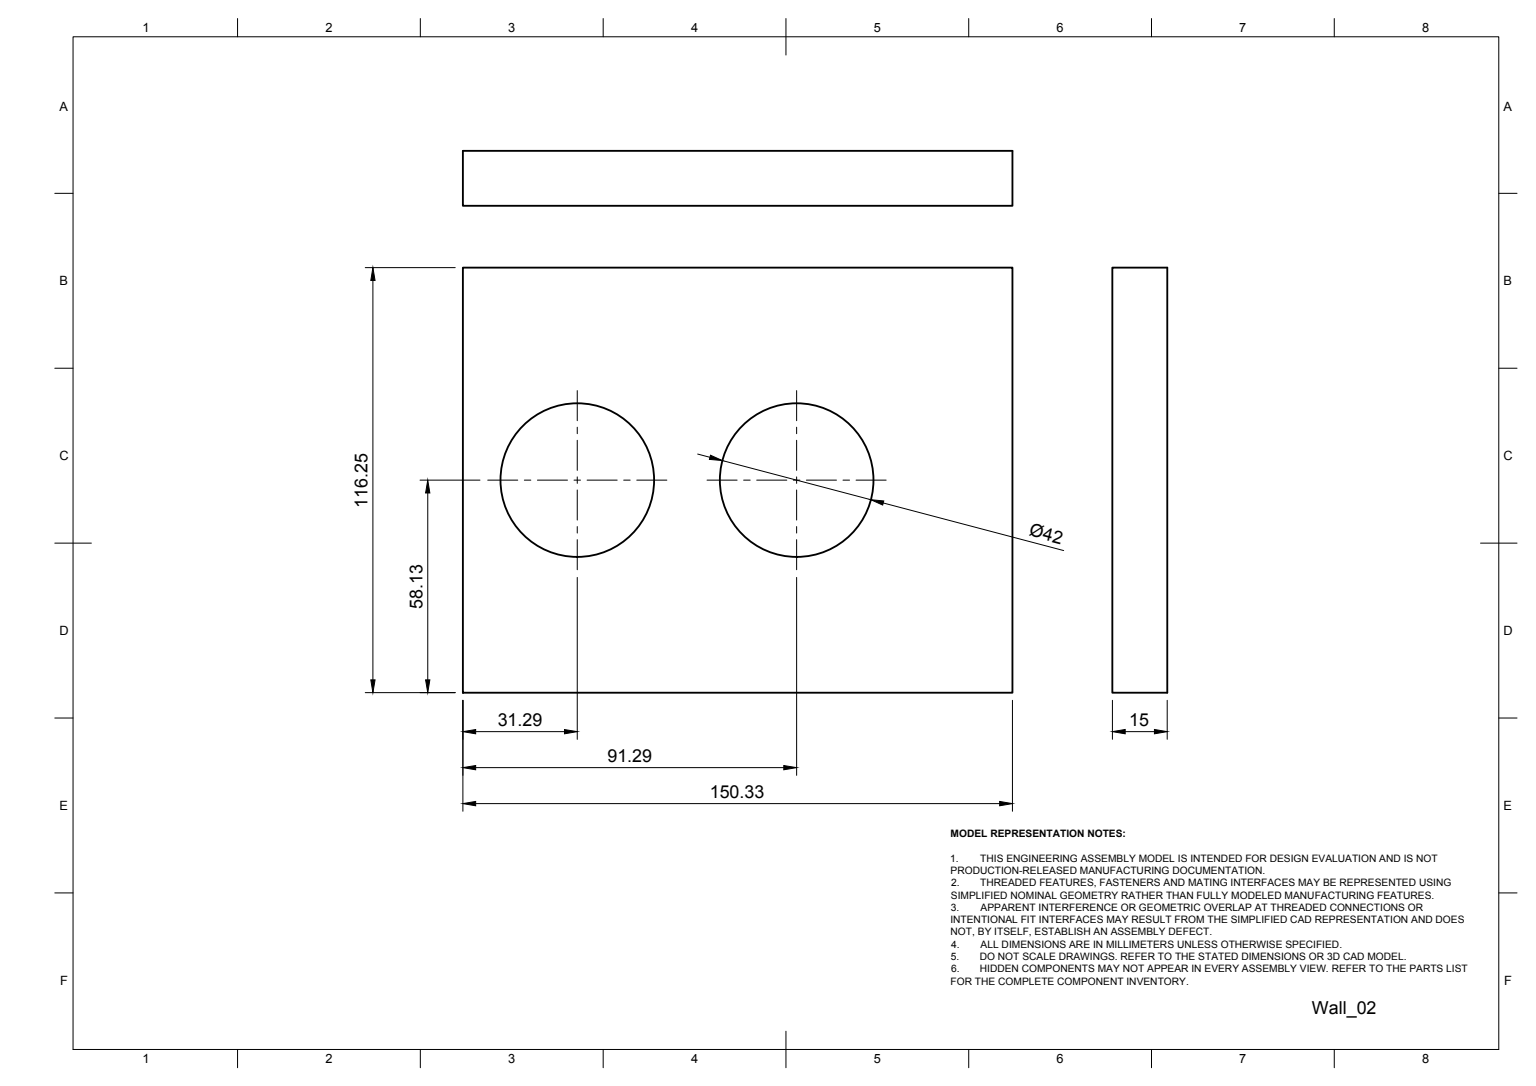
ISO-10303-21;
HEADER;
/* Generated by software containing ST-Developer
 * from STEP Tools, Inc. (www.steptools.com) 
 */

FILE_DESCRIPTION(
/* description */ (''),
/* implementation_level */ '2;1');

FILE_NAME(
/* name */ 'Wall_02.step',
/* time_stamp */ '2026-10-05T21:54:13-07:00',
/* author */ (''),
/* organization */ (''),
/* preprocessor_version */ 'ST-DEVELOPER v20.2',
/* originating_system */ 'Autodesk Translation Framework v15.15.0.0',
/* authorisation */ '');

FILE_SCHEMA (('AUTOMOTIVE_DESIGN { 1 0 10303 214 3 1 1 }'));
ENDSEC;

DATA;
#10=MECHANICAL_DESIGN_GEOMETRIC_PRESENTATION_REPRESENTATION('',(#233),#43781);
#181=SHAPE_REPRESENTATION_RELATIONSHIP('SRR','None',#43819,#189);
#189=ADVANCED_BREP_SHAPE_REPRESENTATION('',(#277),#43779);
#233=STYLED_ITEM('',(#43863),#277);
#277=MANIFOLD_SOLID_BREP('Body1',#13093);
#483=FACE_BOUND('',#2981,.T.);
#484=FACE_BOUND('',#2982,.T.);
#485=FACE_BOUND('',#2985,.T.);
#486=FACE_BOUND('',#2986,.T.);
#1275=PLANE('',#14883);
#1276=PLANE('',#14887);
#1277=PLANE('',#14888);
#1278=PLANE('',#14889);
#1279=PLANE('',#14890);
#1280=PLANE('',#14891);
#2023=FACE_OUTER_BOUND('',#2979,.T.);
#2024=FACE_OUTER_BOUND('',#2980,.T.);
#2025=FACE_OUTER_BOUND('',#2983,.T.);
#2026=FACE_OUTER_BOUND('',#2984,.T.);
#2027=FACE_OUTER_BOUND('',#2987,.T.);
#2028=FACE_OUTER_BOUND('',#2988,.T.);
#2029=FACE_OUTER_BOUND('',#2989,.T.);
#2030=FACE_OUTER_BOUND('',#2990,.T.);
#2979=EDGE_LOOP('',(#11947,#11948,#11949,#11950));
#2980=EDGE_LOOP('',(#11951,#11952,#11953,#11954));
#2981=EDGE_LOOP('',(#11955));
#2982=EDGE_LOOP('',(#11956));
#2983=EDGE_LOOP('',(#11957,#11958,#11959,#11960));
#2984=EDGE_LOOP('',(#11961,#11962,#11963,#11964));
#2985=EDGE_LOOP('',(#11965));
#2986=EDGE_LOOP('',(#11966));
#2987=EDGE_LOOP('',(#11967,#11968,#11969,#11970));
#2988=EDGE_LOOP('',(#11971,#11972,#11973,#11974));
#2989=EDGE_LOOP('',(#11975,#11976,#11977,#11978));
#2990=EDGE_LOOP('',(#11979,#11980,#11981,#11982));
#3423=LINE('',#43681,#3871);
#3424=LINE('',#43686,#3872);
#3425=LINE('',#43688,#3873);
#3426=LINE('',#43690,#3874);
#3427=LINE('',#43691,#3875);
#3428=LINE('',#43696,#3876);
#3429=LINE('',#43701,#3877);
#3430=LINE('',#43703,#3878);
#3431=LINE('',#43705,#3879);
#3432=LINE('',#43706,#3880);
#3433=LINE('',#43708,#3881);
#3434=LINE('',#43709,#3882);
#3435=LINE('',#43711,#3883);
#3436=LINE('',#43713,#3884);
#3871=VECTOR('',#18729,21.);
#3872=VECTOR('',#18734,10.);
#3873=VECTOR('',#18735,10.);
#3874=VECTOR('',#18736,10.);
#3875=VECTOR('',#18737,10.);
#3876=VECTOR('',#18742,21.);
#3877=VECTOR('',#18747,10.);
#3878=VECTOR('',#18748,10.);
#3879=VECTOR('',#18749,10.);
#3880=VECTOR('',#18750,10.);
#3881=VECTOR('',#18753,10.);
#3882=VECTOR('',#18754,10.);
#3883=VECTOR('',#18757,10.);
#3884=VECTOR('',#18760,10.);
#4911=CIRCLE('',#14881,21.);
#4912=CIRCLE('',#14882,21.);
#4913=CIRCLE('',#14884,21.);
#4914=CIRCLE('',#14886,21.);
#6223=VERTEX_POINT('',#43678);
#6224=VERTEX_POINT('',#43680);
#6225=VERTEX_POINT('',#43684);
#6226=VERTEX_POINT('',#43685);
#6227=VERTEX_POINT('',#43687);
#6228=VERTEX_POINT('',#43689);
#6229=VERTEX_POINT('',#43692);
#6230=VERTEX_POINT('',#43695);
#6231=VERTEX_POINT('',#43699);
#6232=VERTEX_POINT('',#43700);
#6233=VERTEX_POINT('',#43702);
#6234=VERTEX_POINT('',#43704);
#8135=EDGE_CURVE('',#6223,#6223,#4911,.T.);
#8136=EDGE_CURVE('',#6223,#6224,#3423,.T.);
#8137=EDGE_CURVE('',#6224,#6224,#4912,.T.);
#8138=EDGE_CURVE('',#6225,#6226,#3424,.T.);
#8139=EDGE_CURVE('',#6227,#6225,#3425,.T.);
#8140=EDGE_CURVE('',#6228,#6227,#3426,.T.);
#8141=EDGE_CURVE('',#6226,#6228,#3427,.T.);
#8142=EDGE_CURVE('',#6229,#6229,#4913,.T.);
#8143=EDGE_CURVE('',#6229,#6230,#3428,.T.);
#8144=EDGE_CURVE('',#6230,#6230,#4914,.T.);
#8145=EDGE_CURVE('',#6231,#6232,#3429,.T.);
#8146=EDGE_CURVE('',#6232,#6233,#3430,.T.);
#8147=EDGE_CURVE('',#6233,#6234,#3431,.T.);
#8148=EDGE_CURVE('',#6234,#6231,#3432,.T.);
#8149=EDGE_CURVE('',#6234,#6227,#3433,.T.);
#8150=EDGE_CURVE('',#6231,#6225,#3434,.T.);
#8151=EDGE_CURVE('',#6232,#6226,#3435,.T.);
#8152=EDGE_CURVE('',#6233,#6228,#3436,.T.);
#11947=ORIENTED_EDGE('',*,*,#8135,.F.);
#11948=ORIENTED_EDGE('',*,*,#8136,.T.);
#11949=ORIENTED_EDGE('',*,*,#8137,.F.);
#11950=ORIENTED_EDGE('',*,*,#8136,.F.);
#11951=ORIENTED_EDGE('',*,*,#8138,.F.);
#11952=ORIENTED_EDGE('',*,*,#8139,.F.);
#11953=ORIENTED_EDGE('',*,*,#8140,.F.);
#11954=ORIENTED_EDGE('',*,*,#8141,.F.);
#11955=ORIENTED_EDGE('',*,*,#8142,.T.);
#11956=ORIENTED_EDGE('',*,*,#8135,.T.);
#11957=ORIENTED_EDGE('',*,*,#8142,.F.);
#11958=ORIENTED_EDGE('',*,*,#8143,.T.);
#11959=ORIENTED_EDGE('',*,*,#8144,.F.);
#11960=ORIENTED_EDGE('',*,*,#8143,.F.);
#11961=ORIENTED_EDGE('',*,*,#8145,.T.);
#11962=ORIENTED_EDGE('',*,*,#8146,.T.);
#11963=ORIENTED_EDGE('',*,*,#8147,.T.);
#11964=ORIENTED_EDGE('',*,*,#8148,.T.);
#11965=ORIENTED_EDGE('',*,*,#8144,.T.);
#11966=ORIENTED_EDGE('',*,*,#8137,.T.);
#11967=ORIENTED_EDGE('',*,*,#8148,.F.);
#11968=ORIENTED_EDGE('',*,*,#8149,.T.);
#11969=ORIENTED_EDGE('',*,*,#8139,.T.);
#11970=ORIENTED_EDGE('',*,*,#8150,.F.);
#11971=ORIENTED_EDGE('',*,*,#8145,.F.);
#11972=ORIENTED_EDGE('',*,*,#8150,.T.);
#11973=ORIENTED_EDGE('',*,*,#8138,.T.);
#11974=ORIENTED_EDGE('',*,*,#8151,.F.);
#11975=ORIENTED_EDGE('',*,*,#8147,.F.);
#11976=ORIENTED_EDGE('',*,*,#8152,.T.);
#11977=ORIENTED_EDGE('',*,*,#8140,.T.);
#11978=ORIENTED_EDGE('',*,*,#8149,.F.);
#11979=ORIENTED_EDGE('',*,*,#8146,.F.);
#11980=ORIENTED_EDGE('',*,*,#8151,.T.);
#11981=ORIENTED_EDGE('',*,*,#8141,.T.);
#11982=ORIENTED_EDGE('',*,*,#8152,.F.);
#12295=CYLINDRICAL_SURFACE('',#14880,21.);
#12296=CYLINDRICAL_SURFACE('',#14885,21.);
#13035=ADVANCED_FACE('',(#2023),#12295,.F.);
#13036=ADVANCED_FACE('',(#2024,#483,#484),#1275,.F.);
#13037=ADVANCED_FACE('',(#2025),#12296,.F.);
#13038=ADVANCED_FACE('',(#2026,#485,#486),#1276,.T.);
#13039=ADVANCED_FACE('',(#2027),#1277,.F.);
#13040=ADVANCED_FACE('',(#2028),#1278,.F.);
#13041=ADVANCED_FACE('',(#2029),#1279,.F.);
#13042=ADVANCED_FACE('',(#2030),#1280,.F.);
#13093=CLOSED_SHELL('',(#13035,#13036,#13037,#13038,#13039,#13040,#13041,
#13042));
#14879=AXIS2_PLACEMENT_3D('',#43676,#18723,#18724);
#14880=AXIS2_PLACEMENT_3D('',#43677,#18725,#18726);
#14881=AXIS2_PLACEMENT_3D('',#43679,#18727,#18728);
#14882=AXIS2_PLACEMENT_3D('',#43682,#18730,#18731);
#14883=AXIS2_PLACEMENT_3D('',#43683,#18732,#18733);
#14884=AXIS2_PLACEMENT_3D('',#43693,#18738,#18739);
#14885=AXIS2_PLACEMENT_3D('',#43694,#18740,#18741);
#14886=AXIS2_PLACEMENT_3D('',#43697,#18743,#18744);
#14887=AXIS2_PLACEMENT_3D('',#43698,#18745,#18746);
#14888=AXIS2_PLACEMENT_3D('',#43707,#18751,#18752);
#14889=AXIS2_PLACEMENT_3D('',#43710,#18755,#18756);
#14890=AXIS2_PLACEMENT_3D('',#43712,#18758,#18759);
#14891=AXIS2_PLACEMENT_3D('',#43714,#18761,#18762);
#18723=DIRECTION('axis',(0.,0.,1.));
#18724=DIRECTION('refdir',(1.,0.,0.));
#18725=DIRECTION('center_axis',(0.,1.,1.28185868640845E-16));
#18726=DIRECTION('ref_axis',(0.,-1.28185868640845E-16,1.));
#18727=DIRECTION('center_axis',(0.,1.,0.));
#18728=DIRECTION('ref_axis',(0.,0.,1.));
#18729=DIRECTION('',(0.,1.,1.28185868640845E-16));
#18730=DIRECTION('center_axis',(0.,-1.,0.));
#18731=DIRECTION('ref_axis',(1.,0.,0.));
#18732=DIRECTION('center_axis',(0.,1.,0.));
#18733=DIRECTION('ref_axis',(0.,0.,1.));
#18734=DIRECTION('',(-1.,0.,0.));
#18735=DIRECTION('',(0.,0.,-1.));
#18736=DIRECTION('',(1.,0.,0.));
#18737=DIRECTION('',(0.,0.,1.));
#18738=DIRECTION('center_axis',(0.,1.,0.));
#18739=DIRECTION('ref_axis',(-1.57772181044206E-30,0.,1.));
#18740=DIRECTION('center_axis',(-3.15544362088403E-30,1.,-1.31112237000141E-14));
#18741=DIRECTION('ref_axis',(-1.57772181044206E-30,1.31112237000141E-14,
1.));
#18742=DIRECTION('',(-3.15544362088403E-30,1.,-1.31112237000141E-14));
#18743=DIRECTION('center_axis',(0.,-1.,0.));
#18744=DIRECTION('ref_axis',(1.,0.,0.));
#18745=DIRECTION('center_axis',(0.,1.,0.));
#18746=DIRECTION('ref_axis',(0.,0.,1.));
#18747=DIRECTION('',(-1.,0.,0.));
#18748=DIRECTION('',(0.,0.,1.));
#18749=DIRECTION('',(1.,0.,0.));
#18750=DIRECTION('',(0.,0.,-1.));
#18751=DIRECTION('center_axis',(-1.,0.,0.));
#18752=DIRECTION('ref_axis',(0.,0.,-1.));
#18753=DIRECTION('',(0.,-1.,0.));
#18754=DIRECTION('',(0.,-1.,0.));
#18755=DIRECTION('center_axis',(0.,0.,1.));
#18756=DIRECTION('ref_axis',(-1.,0.,0.));
#18757=DIRECTION('',(0.,-1.,0.));
#18758=DIRECTION('center_axis',(0.,0.,-1.));
#18759=DIRECTION('ref_axis',(1.,0.,0.));
#18760=DIRECTION('',(0.,-1.,0.));
#18761=DIRECTION('center_axis',(1.,0.,0.));
#18762=DIRECTION('ref_axis',(0.,0.,1.));
#43676=CARTESIAN_POINT('',(0.,0.,0.));
#43677=CARTESIAN_POINT('Origin',(0.,-33.,7.49999756423169));
#43678=CARTESIAN_POINT('',(-2.57175827820944E-15,-45.,-13.5000024357683));
#43679=CARTESIAN_POINT('Origin',(0.,-45.,7.49999756423169));
#43680=CARTESIAN_POINT('',(-2.57175827820944E-15,-30.,-13.5000024357683));
#43681=CARTESIAN_POINT('',(-2.57175827820944E-15,-33.,-13.5000024357683));
#43682=CARTESIAN_POINT('Origin',(0.,-30.,7.49999756423169));
#43683=CARTESIAN_POINT('Origin',(0.,-45.,23.6225292964879));
#43684=CARTESIAN_POINT('',(58.1257387537822,-45.,-51.5400639196098));
#43685=CARTESIAN_POINT('',(-58.1257387537822,-45.,-51.5400639196098));
#43686=CARTESIAN_POINT('',(-58.1257387537822,-45.,-51.5400639196098));
#43687=CARTESIAN_POINT('',(58.1257387537822,-45.,98.7851225125855));
#43688=CARTESIAN_POINT('',(58.1257387537822,-45.,-51.5400639196098));
#43689=CARTESIAN_POINT('',(-58.1257387537822,-45.,98.7851225125855));
#43690=CARTESIAN_POINT('',(58.1257387537822,-45.,98.7851225125855));
#43691=CARTESIAN_POINT('',(-58.1257387537822,-45.,98.7851225125855));
#43692=CARTESIAN_POINT('',(3.70557314396981E-12,-44.9999999999997,46.5000021716098));
#43693=CARTESIAN_POINT('Origin',(3.70814490224802E-12,-44.9999999999994,
67.5000021716098));
#43694=CARTESIAN_POINT('Origin',(3.70814490224802E-12,-33.,67.5000021716096));
#43695=CARTESIAN_POINT('',(3.70557314396981E-12,-30.,46.5000021716096));
#43696=CARTESIAN_POINT('',(3.70557314396981E-12,-33.0000000000003,46.5000021716096));
#43697=CARTESIAN_POINT('Origin',(3.70814490224802E-12,-30.,67.5000021716098));
#43698=CARTESIAN_POINT('Origin',(0.,-30.,23.6225292964879));
#43699=CARTESIAN_POINT('',(58.1257387537822,-30.,-51.5400639196098));
#43700=CARTESIAN_POINT('',(-58.1257387537822,-30.,-51.5400639196098));
#43701=CARTESIAN_POINT('',(29.0628693768911,-30.,-51.5400639196098));
#43702=CARTESIAN_POINT('',(-58.1257387537822,-30.,98.7851225125855));
#43703=CARTESIAN_POINT('',(-58.1257387537822,-30.,-13.958767311561));
#43704=CARTESIAN_POINT('',(58.1257387537822,-30.,98.7851225125855));
#43705=CARTESIAN_POINT('',(-29.0628693768911,-30.,98.7851225125855));
#43706=CARTESIAN_POINT('',(58.1257387537822,-30.,61.2038259045367));
#43707=CARTESIAN_POINT('Origin',(58.1257387537822,5.,98.7851225125855));
#43708=CARTESIAN_POINT('',(58.1257387537822,5.,98.7851225125855));
#43709=CARTESIAN_POINT('',(58.1257387537822,5.,-51.5400639196098));
#43710=CARTESIAN_POINT('Origin',(58.1257387537822,5.,-51.5400639196098));
#43711=CARTESIAN_POINT('',(-58.1257387537822,5.,-51.5400639196098));
#43712=CARTESIAN_POINT('Origin',(-58.1257387537822,5.,98.7851225125855));
#43713=CARTESIAN_POINT('',(-58.1257387537822,5.,98.7851225125855));
#43714=CARTESIAN_POINT('Origin',(-58.1257387537822,5.,-51.5400639196098));
#43769=UNCERTAINTY_MEASURE_WITH_UNIT(LENGTH_MEASURE(0.01),#43782,
'DISTANCE_ACCURACY_VALUE',
'Maximum model space distance between geometric entities at asserted c
onnectivities');
#43771=UNCERTAINTY_MEASURE_WITH_UNIT(LENGTH_MEASURE(0.01),#43782,
'DISTANCE_ACCURACY_VALUE',
'Maximum model space distance between geometric entities at asserted c
onnectivities');
#43779=(
GEOMETRIC_REPRESENTATION_CONTEXT(3)
GLOBAL_UNCERTAINTY_ASSIGNED_CONTEXT((#43769))
GLOBAL_UNIT_ASSIGNED_CONTEXT((#43782,#43784,#43785))
REPRESENTATION_CONTEXT('','3D')
);
#43781=(
GEOMETRIC_REPRESENTATION_CONTEXT(3)
GLOBAL_UNCERTAINTY_ASSIGNED_CONTEXT((#43771))
GLOBAL_UNIT_ASSIGNED_CONTEXT((#43782,#43784,#43785))
REPRESENTATION_CONTEXT('','3D')
);
#43782=(
LENGTH_UNIT()
NAMED_UNIT(*)
SI_UNIT(.MILLI.,.METRE.)
);
#43784=(
NAMED_UNIT(*)
PLANE_ANGLE_UNIT()
SI_UNIT($,.RADIAN.)
);
#43785=(
NAMED_UNIT(*)
SI_UNIT($,.STERADIAN.)
SOLID_ANGLE_UNIT()
);
#43793=SHAPE_DEFINITION_REPRESENTATION(#43802,#43819);
#43802=PRODUCT_DEFINITION_SHAPE('',$,#43829);
#43819=SHAPE_REPRESENTATION('',(#14879),#43779);
#43821=PRODUCT_DEFINITION_CONTEXT('part definition',#43850,'design');
#43829=PRODUCT_DEFINITION('Wall_02','Wall_02',#43838,#43821);
#43838=PRODUCT_DEFINITION_FORMATION('',$,#43859);
#43850=APPLICATION_CONTEXT(
'Core Data for Automotive Mechanical Design Process');
#43851=PRODUCT_CONTEXT('part definition',#43850,'mechanical');
#43859=PRODUCT('Wall_02','Wall_02',$,(#43851));
#43863=PRESENTATION_STYLE_ASSIGNMENT((#43866));
#43866=SURFACE_STYLE_USAGE(.BOTH.,#43869);
#43869=SURFACE_SIDE_STYLE('',(#43872));
#43872=SURFACE_STYLE_FILL_AREA(#43875);
#43875=FILL_AREA_STYLE('Opaque(160,160,160)',(#43878));
#43878=FILL_AREA_STYLE_COLOUR('Opaque(160,160,160)',#43881);
#43881=COLOUR_RGB('Opaque(160,160,160)', 0.31764706, 0.68627451, 0.89019608);
ENDSEC;
END-ISO-10303-21;
